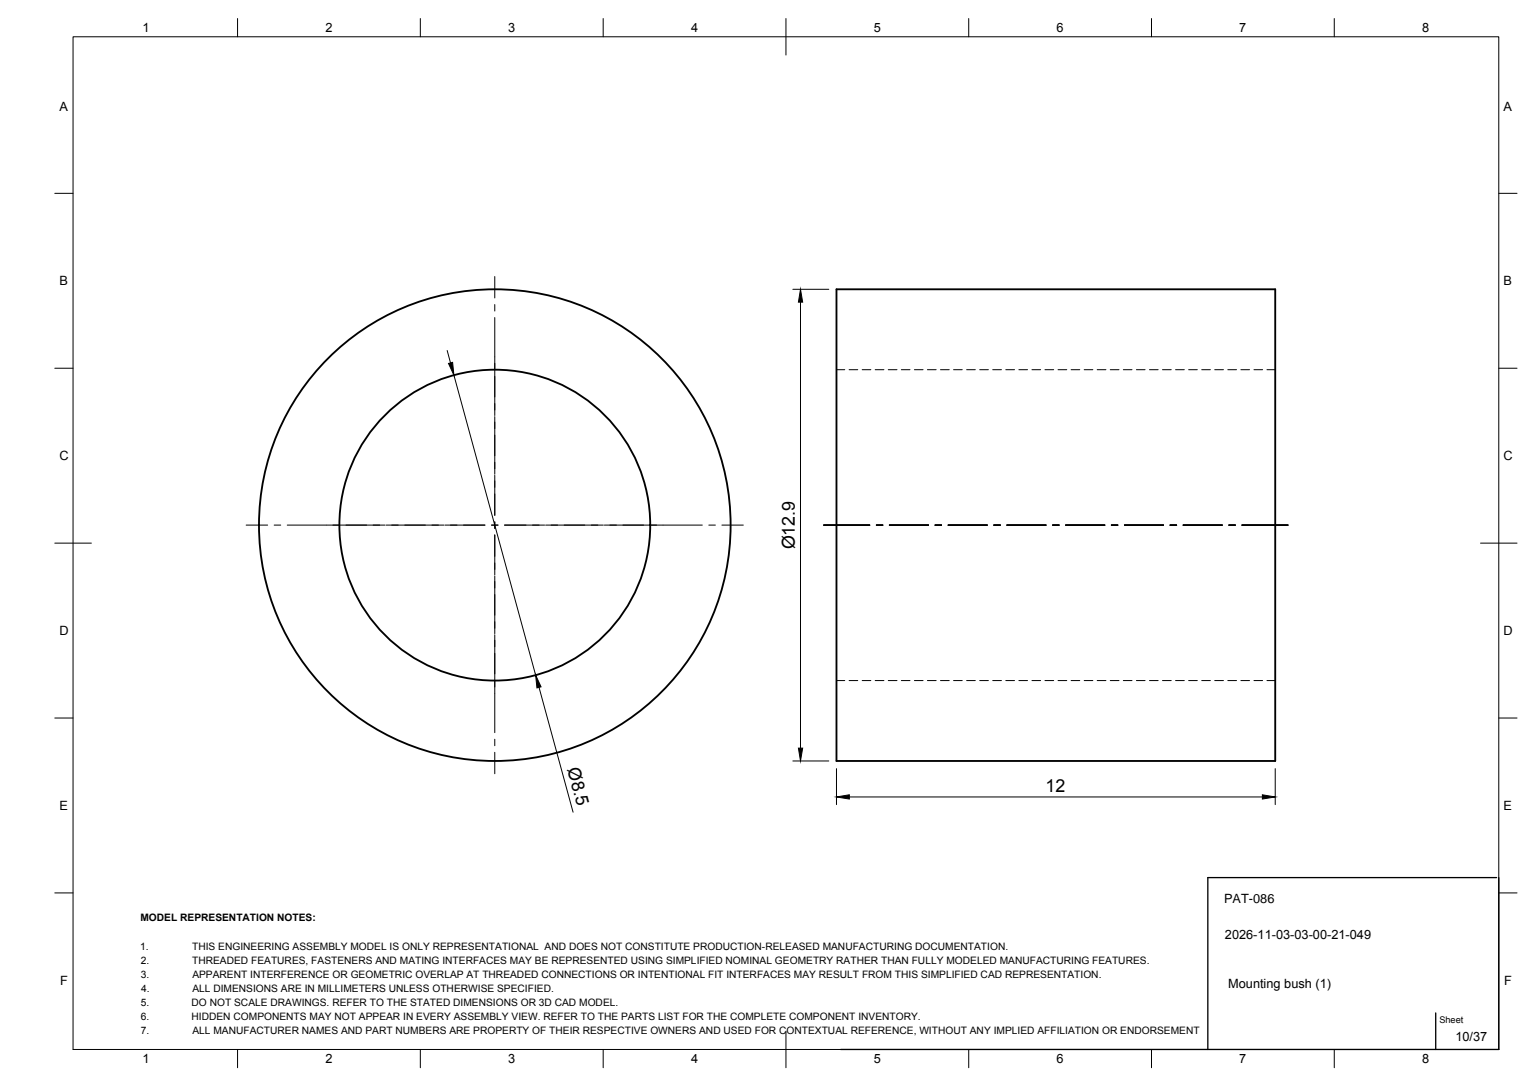
ISO-10303-21;
HEADER;
/* Generated by software containing ST-Developer
 * from STEP Tools, Inc. (www.steptools.com) 
 */

FILE_DESCRIPTION(
/* description */ ('Ratchet and pawl hand winch drum'),
/* implementation_level */ '2;1');

FILE_NAME(
/* name */ 'Mounting bush (1).step',
/* time_stamp */ '2026-10-27T12:42:58-07:00',
/* author */ (''),
/* organization */ (''),
/* preprocessor_version */ 'ST-DEVELOPER v20.2',
/* originating_system */ 'Autodesk Translation Framework v15.17.0.0',
/* authorisation */ '');

FILE_SCHEMA (('AUTOMOTIVE_DESIGN { 1 0 10303 214 3 1 1 }'));
ENDSEC;

DATA;
#10=MECHANICAL_DESIGN_GEOMETRIC_PRESENTATION_REPRESENTATION('',(#394),#11801);
#326=SHAPE_REPRESENTATION_RELATIONSHIP('SRR','None',#11952,#360);
#360=ADVANCED_BREP_SHAPE_REPRESENTATION('',(#429),#11769);
#394=STYLED_ITEM('',(#12206),#429);
#429=MANIFOLD_SOLID_BREP('Body1',#6271);
#494=FACE_BOUND('',#1289,.T.);
#495=FACE_BOUND('',#1291,.T.);
#631=PLANE('',#6789);
#632=PLANE('',#6790);
#892=FACE_OUTER_BOUND('',#1286,.T.);
#893=FACE_OUTER_BOUND('',#1287,.T.);
#894=FACE_OUTER_BOUND('',#1288,.T.);
#895=FACE_OUTER_BOUND('',#1290,.T.);
#1286=EDGE_LOOP('',(#4475,#4476,#4477,#4478));
#1287=EDGE_LOOP('',(#4479,#4480,#4481,#4482));
#1288=EDGE_LOOP('',(#4483));
#1289=EDGE_LOOP('',(#4484));
#1290=EDGE_LOOP('',(#4485));
#1291=EDGE_LOOP('',(#4486));
#1767=LINE('',#9481,#2278);
#1768=LINE('',#9487,#2279);
#2278=VECTOR('',#7640,0.425);
#2279=VECTOR('',#7647,0.645);
#2763=CIRCLE('',#6784,0.425);
#2764=CIRCLE('',#6785,0.425);
#2765=CIRCLE('',#6787,0.645);
#2766=CIRCLE('',#6788,0.645);
#3018=VERTEX_POINT('',#9478);
#3019=VERTEX_POINT('',#9480);
#3020=VERTEX_POINT('',#9484);
#3021=VERTEX_POINT('',#9486);
#3581=EDGE_CURVE('',#3018,#3018,#2763,.T.);
#3582=EDGE_CURVE('',#3018,#3019,#1767,.T.);
#3583=EDGE_CURVE('',#3019,#3019,#2764,.T.);
#3584=EDGE_CURVE('',#3020,#3020,#2765,.T.);
#3585=EDGE_CURVE('',#3020,#3021,#1768,.T.);
#3586=EDGE_CURVE('',#3021,#3021,#2766,.T.);
#4475=ORIENTED_EDGE('',*,*,#3581,.F.);
#4476=ORIENTED_EDGE('',*,*,#3582,.T.);
#4477=ORIENTED_EDGE('',*,*,#3583,.T.);
#4478=ORIENTED_EDGE('',*,*,#3582,.F.);
#4479=ORIENTED_EDGE('',*,*,#3584,.F.);
#4480=ORIENTED_EDGE('',*,*,#3585,.T.);
#4481=ORIENTED_EDGE('',*,*,#3586,.T.);
#4482=ORIENTED_EDGE('',*,*,#3585,.F.);
#4483=ORIENTED_EDGE('',*,*,#3584,.T.);
#4484=ORIENTED_EDGE('',*,*,#3581,.T.);
#4485=ORIENTED_EDGE('',*,*,#3586,.F.);
#4486=ORIENTED_EDGE('',*,*,#3583,.F.);
#5829=CYLINDRICAL_SURFACE('',#6783,0.425);
#5830=CYLINDRICAL_SURFACE('',#6786,0.645);
#5962=ADVANCED_FACE('',(#892),#5829,.F.);
#5963=ADVANCED_FACE('',(#893),#5830,.T.);
#5964=ADVANCED_FACE('',(#894,#494),#631,.T.);
#5965=ADVANCED_FACE('',(#895,#495),#632,.F.);
#6271=CLOSED_SHELL('',(#5962,#5963,#5964,#5965));
#6782=AXIS2_PLACEMENT_3D('',#9476,#7634,#7635);
#6783=AXIS2_PLACEMENT_3D('',#9477,#7636,#7637);
#6784=AXIS2_PLACEMENT_3D('',#9479,#7638,#7639);
#6785=AXIS2_PLACEMENT_3D('',#9482,#7641,#7642);
#6786=AXIS2_PLACEMENT_3D('',#9483,#7643,#7644);
#6787=AXIS2_PLACEMENT_3D('',#9485,#7645,#7646);
#6788=AXIS2_PLACEMENT_3D('',#9488,#7648,#7649);
#6789=AXIS2_PLACEMENT_3D('',#9489,#7650,#7651);
#6790=AXIS2_PLACEMENT_3D('',#9490,#7652,#7653);
#7634=DIRECTION('axis',(0.,0.,1.));
#7635=DIRECTION('refdir',(1.,0.,0.));
#7636=DIRECTION('center_axis',(0.,0.,1.));
#7637=DIRECTION('ref_axis',(1.,0.,0.));
#7638=DIRECTION('center_axis',(0.,0.,-1.));
#7639=DIRECTION('ref_axis',(1.,0.,0.));
#7640=DIRECTION('',(0.,0.,-1.));
#7641=DIRECTION('center_axis',(0.,0.,-1.));
#7642=DIRECTION('ref_axis',(1.,0.,0.));
#7643=DIRECTION('center_axis',(0.,0.,1.));
#7644=DIRECTION('ref_axis',(1.,0.,0.));
#7645=DIRECTION('center_axis',(0.,0.,1.));
#7646=DIRECTION('ref_axis',(1.,0.,0.));
#7647=DIRECTION('',(0.,0.,-1.));
#7648=DIRECTION('center_axis',(0.,0.,1.));
#7649=DIRECTION('ref_axis',(1.,0.,0.));
#7650=DIRECTION('center_axis',(0.,0.,1.));
#7651=DIRECTION('ref_axis',(1.,0.,0.));
#7652=DIRECTION('center_axis',(0.,0.,1.));
#7653=DIRECTION('ref_axis',(1.,0.,0.));
#9476=CARTESIAN_POINT('',(0.,0.,0.));
#9477=CARTESIAN_POINT('Origin',(4.75,0.,3.2));
#9478=CARTESIAN_POINT('',(4.325,-5.20474889637625E-17,4.4));
#9479=CARTESIAN_POINT('Origin',(4.75,0.,4.4));
#9480=CARTESIAN_POINT('',(4.325,-5.20474889637625E-17,3.2));
#9481=CARTESIAN_POINT('',(4.325,-5.20474889637625E-17,3.2));
#9482=CARTESIAN_POINT('Origin',(4.75,0.,3.2));
#9483=CARTESIAN_POINT('Origin',(4.75,0.,3.2));
#9484=CARTESIAN_POINT('',(4.105,-7.89897185450042E-17,4.4));
#9485=CARTESIAN_POINT('Origin',(4.75,0.,4.4));
#9486=CARTESIAN_POINT('',(4.105,-7.89897185450042E-17,3.2));
#9487=CARTESIAN_POINT('',(4.105,-7.89897185450042E-17,3.2));
#9488=CARTESIAN_POINT('Origin',(4.75,0.,3.2));
#9489=CARTESIAN_POINT('Origin',(4.75,0.,4.4));
#9490=CARTESIAN_POINT('Origin',(4.75,0.,3.2));
#11729=UNCERTAINTY_MEASURE_WITH_UNIT(LENGTH_MEASURE(0.001),#11802,
'DISTANCE_ACCURACY_VALUE',
'Maximum model space distance between geometric entities at asserted c
onnectivities');
#11761=UNCERTAINTY_MEASURE_WITH_UNIT(LENGTH_MEASURE(0.001),#11802,
'DISTANCE_ACCURACY_VALUE',
'Maximum model space distance between geometric entities at asserted c
onnectivities');
#11769=(
GEOMETRIC_REPRESENTATION_CONTEXT(3)
GLOBAL_UNCERTAINTY_ASSIGNED_CONTEXT((#11729))
GLOBAL_UNIT_ASSIGNED_CONTEXT((#11802,#11804,#11805))
REPRESENTATION_CONTEXT('','3D')
);
#11801=(
GEOMETRIC_REPRESENTATION_CONTEXT(3)
GLOBAL_UNCERTAINTY_ASSIGNED_CONTEXT((#11761))
GLOBAL_UNIT_ASSIGNED_CONTEXT((#11802,#11804,#11805))
REPRESENTATION_CONTEXT('','3D')
);
#11802=(
LENGTH_UNIT()
NAMED_UNIT(*)
SI_UNIT(.CENTI.,.METRE.)
);
#11804=(
NAMED_UNIT(*)
PLANE_ANGLE_UNIT()
SI_UNIT($,.RADIAN.)
);
#11805=(
NAMED_UNIT(*)
SI_UNIT($,.STERADIAN.)
SOLID_ANGLE_UNIT()
);
#11813=SHAPE_DEFINITION_REPRESENTATION(#11852,#11952);
#11852=PRODUCT_DEFINITION_SHAPE('',$,#11992);
#11952=SHAPE_REPRESENTATION('',(#6782),#11769);
#11984=PRODUCT_DEFINITION_CONTEXT('part definition',#12103,'design');
#11992=PRODUCT_DEFINITION('Mounting bush (1)','Mounting bush (1)',#12031,
#11984);
#12031=PRODUCT_DEFINITION_FORMATION('',$,#12112);
#12103=APPLICATION_CONTEXT(
'Core Data for Automotive Mechanical Design Process');
#12104=PRODUCT_CONTEXT('part definition',#12103,'mechanical');
#12112=PRODUCT('Mounting bush (1)','Mounting bush (1)','Mounting bush (1)',(#12104));
#12200=COLOUR_RGB('Sky Blue',0.24,0.69,0.87);
#12201=FILL_AREA_STYLE_COLOUR('',#12200);
#12202=FILL_AREA_STYLE('',(#12201));
#12203=SURFACE_STYLE_FILL_AREA(#12202);
#12204=SURFACE_SIDE_STYLE('',(#12203));
#12205=SURFACE_STYLE_USAGE(.BOTH.,#12204);
#12206=PRESENTATION_STYLE_ASSIGNMENT((#12205));
ENDSEC;
END-ISO-10303-21;
